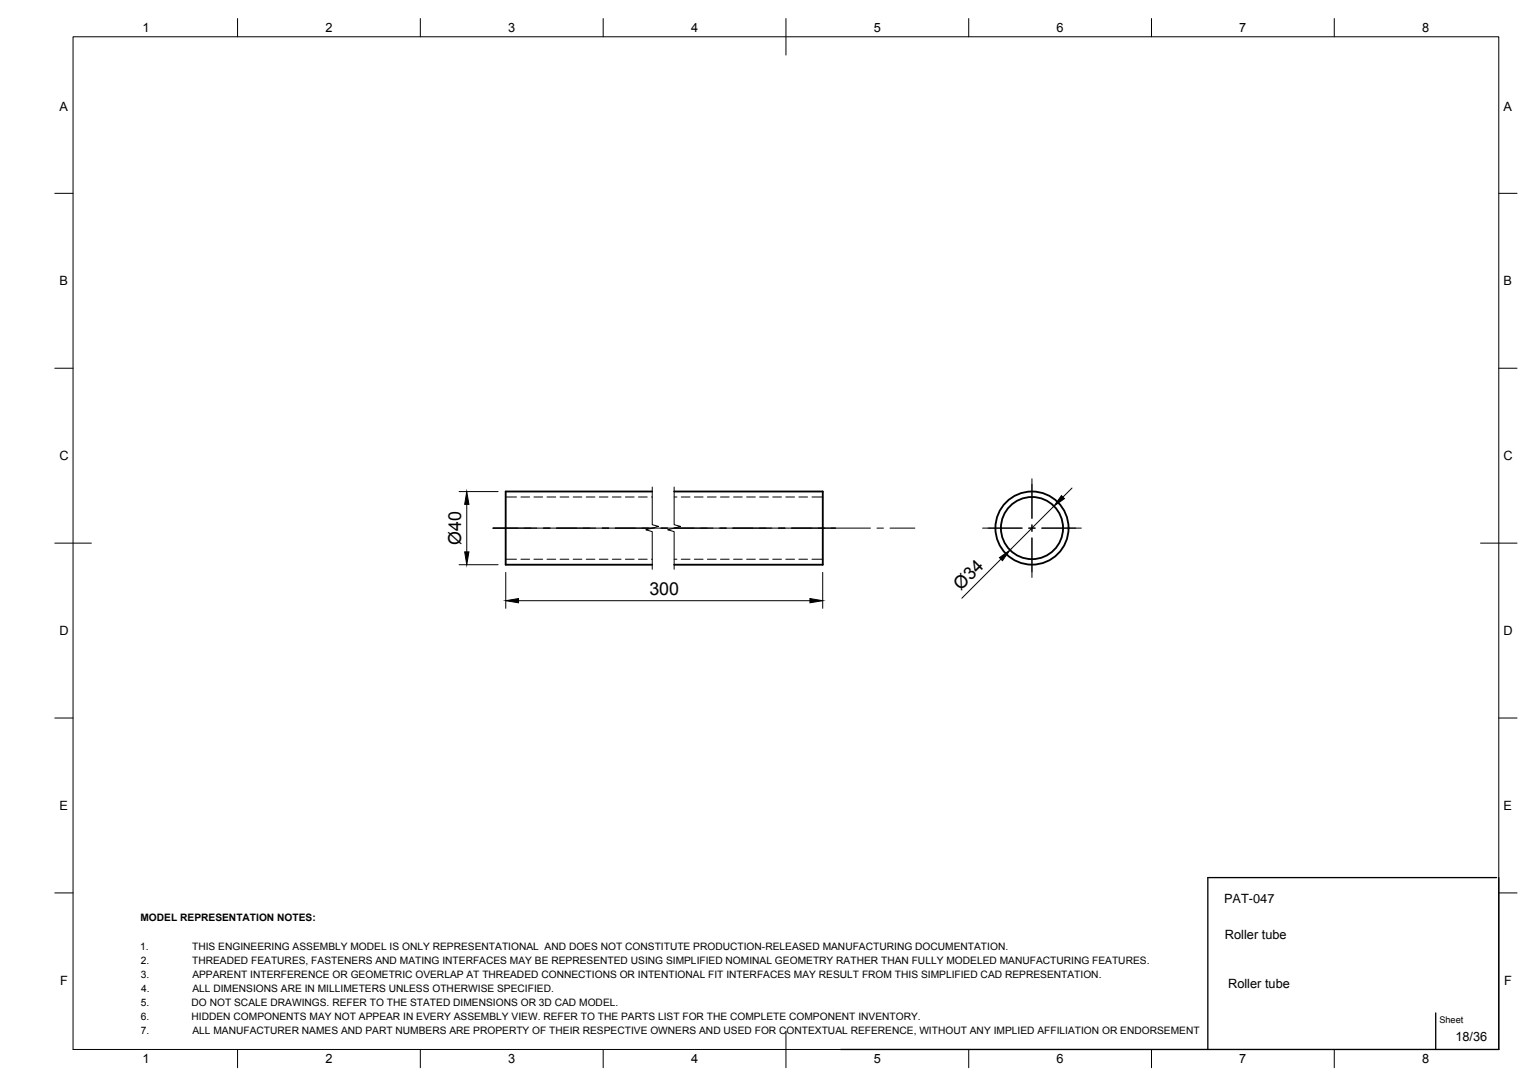
ISO-10303-21;
HEADER;
/* Generated by software containing ST-Developer
 * from STEP Tools, Inc. (www.steptools.com) 
 */

FILE_DESCRIPTION(
/* description */ ('Gravity roller conveyor section'),
/* implementation_level */ '2;1');

FILE_NAME(
/* name */ 'Roller tube.step',
/* time_stamp */ '2026-11-02T07:43:02-08:00',
/* author */ (''),
/* organization */ (''),
/* preprocessor_version */ 'ST-DEVELOPER v20.2',
/* originating_system */ 'Autodesk Translation Framework v15.17.0.0',
/* authorisation */ '');

FILE_SCHEMA (('AUTOMOTIVE_DESIGN { 1 0 10303 214 3 1 1 }'));
ENDSEC;

DATA;
#10=MECHANICAL_DESIGN_GEOMETRIC_PRESENTATION_REPRESENTATION('',(#543),#13821);
#475=SHAPE_REPRESENTATION_RELATIONSHIP('SRR','None',#14013,#509);
#509=ADVANCED_BREP_SHAPE_REPRESENTATION('',(#583),#13800);
#543=STYLED_ITEM('',(#14192),#583);
#583=MANIFOLD_SOLID_BREP('Body1',#7643);
#650=FACE_BOUND('',#1715,.T.);
#651=FACE_BOUND('',#1717,.T.);
#913=PLANE('',#8373);
#914=PLANE('',#8374);
#1252=FACE_OUTER_BOUND('',#1712,.T.);
#1253=FACE_OUTER_BOUND('',#1713,.T.);
#1254=FACE_OUTER_BOUND('',#1714,.T.);
#1255=FACE_OUTER_BOUND('',#1716,.T.);
#1712=EDGE_LOOP('',(#6462,#6463,#6464,#6465));
#1713=EDGE_LOOP('',(#6466,#6467,#6468,#6469));
#1714=EDGE_LOOP('',(#6470));
#1715=EDGE_LOOP('',(#6471));
#1716=EDGE_LOOP('',(#6472));
#1717=EDGE_LOOP('',(#6473));
#2502=LINE('',#12558,#3220);
#2503=LINE('',#12564,#3221);
#3220=VECTOR('',#10023,1.7);
#3221=VECTOR('',#10030,2.);
#3430=CIRCLE('',#8368,1.7);
#3431=CIRCLE('',#8369,1.7);
#3432=CIRCLE('',#8371,2.);
#3433=CIRCLE('',#8372,2.);
#4008=VERTEX_POINT('',#12555);
#4009=VERTEX_POINT('',#12557);
#4010=VERTEX_POINT('',#12561);
#4011=VERTEX_POINT('',#12563);
#4868=EDGE_CURVE('',#4008,#4008,#3430,.T.);
#4869=EDGE_CURVE('',#4008,#4009,#2502,.T.);
#4870=EDGE_CURVE('',#4009,#4009,#3431,.T.);
#4871=EDGE_CURVE('',#4010,#4010,#3432,.T.);
#4872=EDGE_CURVE('',#4010,#4011,#2503,.T.);
#4873=EDGE_CURVE('',#4011,#4011,#3433,.T.);
#6462=ORIENTED_EDGE('',*,*,#4868,.F.);
#6463=ORIENTED_EDGE('',*,*,#4869,.T.);
#6464=ORIENTED_EDGE('',*,*,#4870,.T.);
#6465=ORIENTED_EDGE('',*,*,#4869,.F.);
#6466=ORIENTED_EDGE('',*,*,#4871,.F.);
#6467=ORIENTED_EDGE('',*,*,#4872,.T.);
#6468=ORIENTED_EDGE('',*,*,#4873,.T.);
#6469=ORIENTED_EDGE('',*,*,#4872,.F.);
#6470=ORIENTED_EDGE('',*,*,#4871,.T.);
#6471=ORIENTED_EDGE('',*,*,#4868,.T.);
#6472=ORIENTED_EDGE('',*,*,#4873,.F.);
#6473=ORIENTED_EDGE('',*,*,#4870,.F.);
#7156=CYLINDRICAL_SURFACE('',#8367,1.7);
#7157=CYLINDRICAL_SURFACE('',#8370,2.);
#7453=ADVANCED_FACE('',(#1252),#7156,.F.);
#7454=ADVANCED_FACE('',(#1253),#7157,.T.);
#7455=ADVANCED_FACE('',(#1254,#650),#913,.T.);
#7456=ADVANCED_FACE('',(#1255,#651),#914,.F.);
#7643=CLOSED_SHELL('',(#7453,#7454,#7455,#7456));
#8366=AXIS2_PLACEMENT_3D('',#12553,#10017,#10018);
#8367=AXIS2_PLACEMENT_3D('',#12554,#10019,#10020);
#8368=AXIS2_PLACEMENT_3D('',#12556,#10021,#10022);
#8369=AXIS2_PLACEMENT_3D('',#12559,#10024,#10025);
#8370=AXIS2_PLACEMENT_3D('',#12560,#10026,#10027);
#8371=AXIS2_PLACEMENT_3D('',#12562,#10028,#10029);
#8372=AXIS2_PLACEMENT_3D('',#12565,#10031,#10032);
#8373=AXIS2_PLACEMENT_3D('',#12566,#10033,#10034);
#8374=AXIS2_PLACEMENT_3D('',#12567,#10035,#10036);
#10017=DIRECTION('axis',(0.,0.,1.));
#10018=DIRECTION('refdir',(1.,0.,0.));
#10019=DIRECTION('center_axis',(0.,1.,0.));
#10020=DIRECTION('ref_axis',(1.,0.,0.));
#10021=DIRECTION('center_axis',(0.,-1.,0.));
#10022=DIRECTION('ref_axis',(1.,0.,0.));
#10023=DIRECTION('',(0.,-1.,0.));
#10024=DIRECTION('center_axis',(0.,-1.,0.));
#10025=DIRECTION('ref_axis',(1.,0.,0.));
#10026=DIRECTION('center_axis',(0.,1.,0.));
#10027=DIRECTION('ref_axis',(1.,0.,0.));
#10028=DIRECTION('center_axis',(0.,1.,0.));
#10029=DIRECTION('ref_axis',(1.,0.,0.));
#10030=DIRECTION('',(0.,-1.,0.));
#10031=DIRECTION('center_axis',(0.,1.,0.));
#10032=DIRECTION('ref_axis',(1.,0.,0.));
#10033=DIRECTION('center_axis',(0.,1.,0.));
#10034=DIRECTION('ref_axis',(1.,0.,0.));
#10035=DIRECTION('center_axis',(0.,1.,0.));
#10036=DIRECTION('ref_axis',(1.,0.,0.));
#12553=CARTESIAN_POINT('',(0.,0.,0.));
#12554=CARTESIAN_POINT('Origin',(3.,0.,8.));
#12555=CARTESIAN_POINT('',(1.3,30.,8.));
#12556=CARTESIAN_POINT('Origin',(3.,30.,8.));
#12557=CARTESIAN_POINT('',(1.3,0.,8.));
#12558=CARTESIAN_POINT('',(1.3,0.,8.));
#12559=CARTESIAN_POINT('Origin',(3.,0.,8.));
#12560=CARTESIAN_POINT('Origin',(3.,0.,8.));
#12561=CARTESIAN_POINT('',(1.,30.,8.));
#12562=CARTESIAN_POINT('Origin',(3.,30.,8.));
#12563=CARTESIAN_POINT('',(1.,0.,8.));
#12564=CARTESIAN_POINT('',(1.,0.,8.));
#12565=CARTESIAN_POINT('Origin',(3.,0.,8.));
#12566=CARTESIAN_POINT('Origin',(3.,30.,8.));
#12567=CARTESIAN_POINT('Origin',(3.,0.,8.));
#13761=UNCERTAINTY_MEASURE_WITH_UNIT(LENGTH_MEASURE(0.001),#13822,
'DISTANCE_ACCURACY_VALUE',
'Maximum model space distance between geometric entities at asserted c
onnectivities');
#13782=UNCERTAINTY_MEASURE_WITH_UNIT(LENGTH_MEASURE(0.001),#13822,
'DISTANCE_ACCURACY_VALUE',
'Maximum model space distance between geometric entities at asserted c
onnectivities');
#13800=(
GEOMETRIC_REPRESENTATION_CONTEXT(3)
GLOBAL_UNCERTAINTY_ASSIGNED_CONTEXT((#13761))
GLOBAL_UNIT_ASSIGNED_CONTEXT((#13822,#13824,#13825))
REPRESENTATION_CONTEXT('','3D')
);
#13821=(
GEOMETRIC_REPRESENTATION_CONTEXT(3)
GLOBAL_UNCERTAINTY_ASSIGNED_CONTEXT((#13782))
GLOBAL_UNIT_ASSIGNED_CONTEXT((#13822,#13824,#13825))
REPRESENTATION_CONTEXT('','3D')
);
#13822=(
LENGTH_UNIT()
NAMED_UNIT(*)
SI_UNIT(.CENTI.,.METRE.)
);
#13824=(
NAMED_UNIT(*)
PLANE_ANGLE_UNIT()
SI_UNIT($,.RADIAN.)
);
#13825=(
NAMED_UNIT(*)
SI_UNIT($,.STERADIAN.)
SOLID_ANGLE_UNIT()
);
#13843=SHAPE_DEFINITION_REPRESENTATION(#13881,#14013);
#13881=PRODUCT_DEFINITION_SHAPE('',$,#14052);
#14013=SHAPE_REPRESENTATION('',(#8366),#13800);
#14034=PRODUCT_DEFINITION_CONTEXT('part definition',#14150,'design');
#14052=PRODUCT_DEFINITION('Roller tube','Roller tube',#14090,#14034);
#14090=PRODUCT_DEFINITION_FORMATION('',$,#14169);
#14150=APPLICATION_CONTEXT(
'Core Data for Automotive Mechanical Design Process');
#14151=PRODUCT_CONTEXT('part definition',#14150,'mechanical');
#14169=PRODUCT('Roller tube','Roller tube','Roller tube',(#14151));
#14192=PRESENTATION_STYLE_ASSIGNMENT((#14197));
#14197=SURFACE_STYLE_USAGE(.BOTH.,#14202);
#14202=SURFACE_SIDE_STYLE('',(#14207));
#14207=SURFACE_STYLE_FILL_AREA(#14212);
#14212=FILL_AREA_STYLE('CAD Library Painted - Engineering blue',(#14217));
#14217=FILL_AREA_STYLE_COLOUR('CAD Library Painted - Engineering blue',
#14222);
#14222=COLOUR_RGB('CAD Library Painted - Engineering blue',0.12156862745098,
0.356862745098039,0.6);
ENDSEC;
END-ISO-10303-21;
